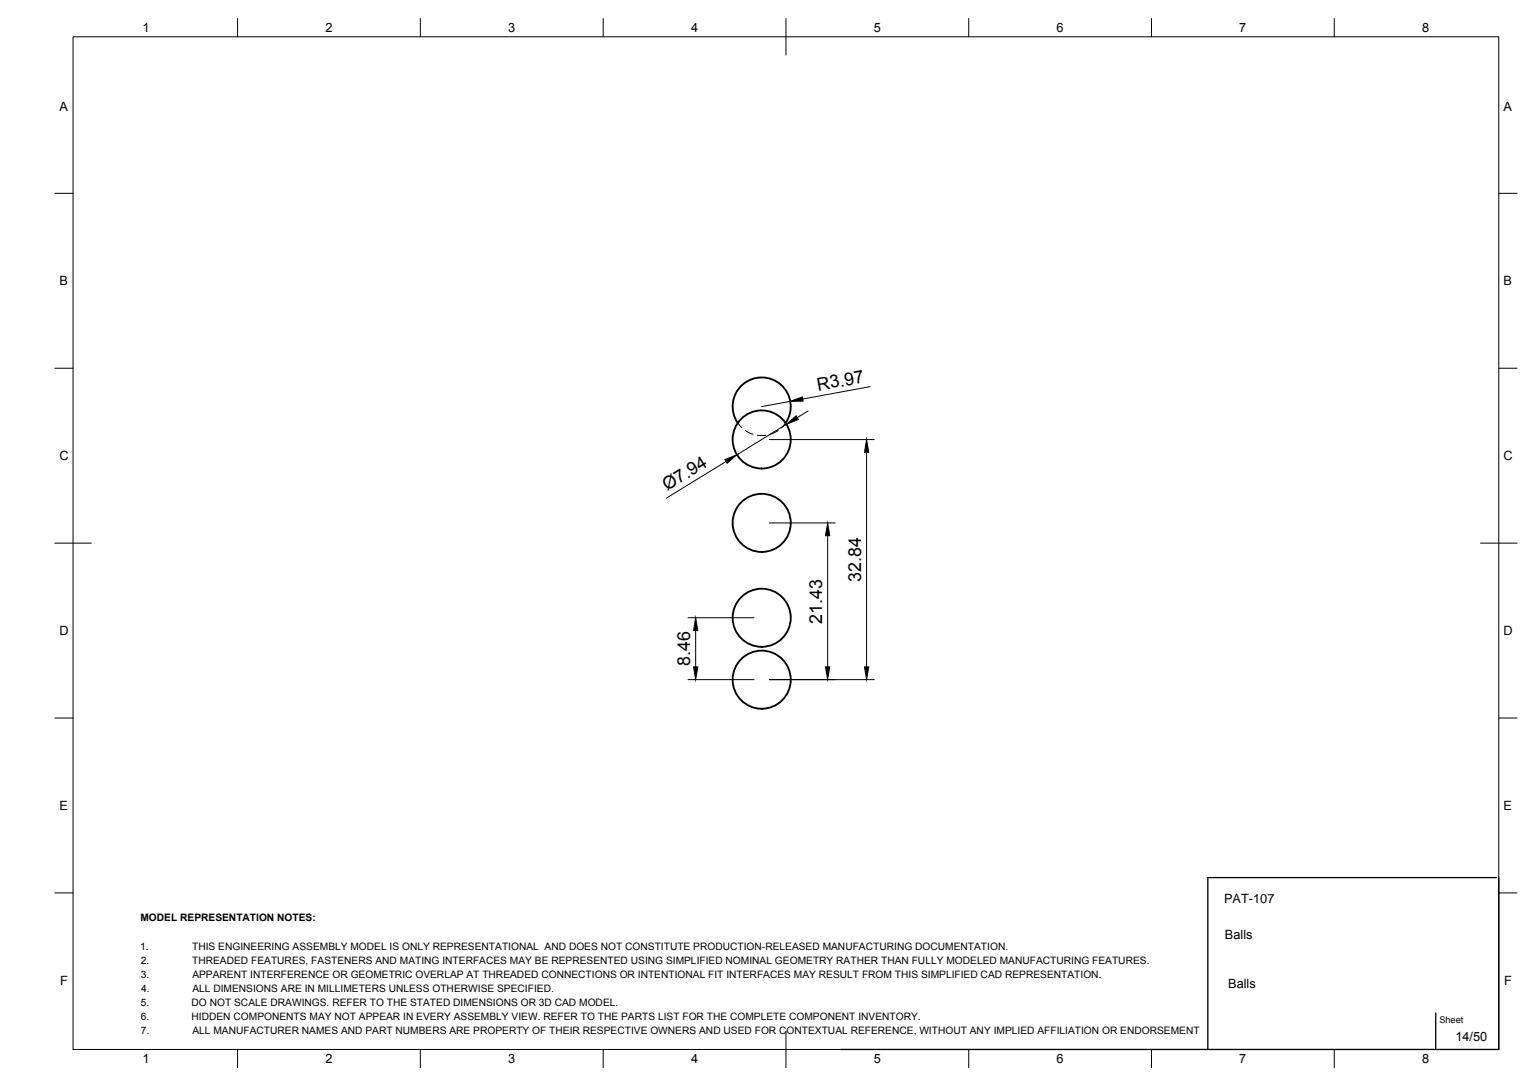
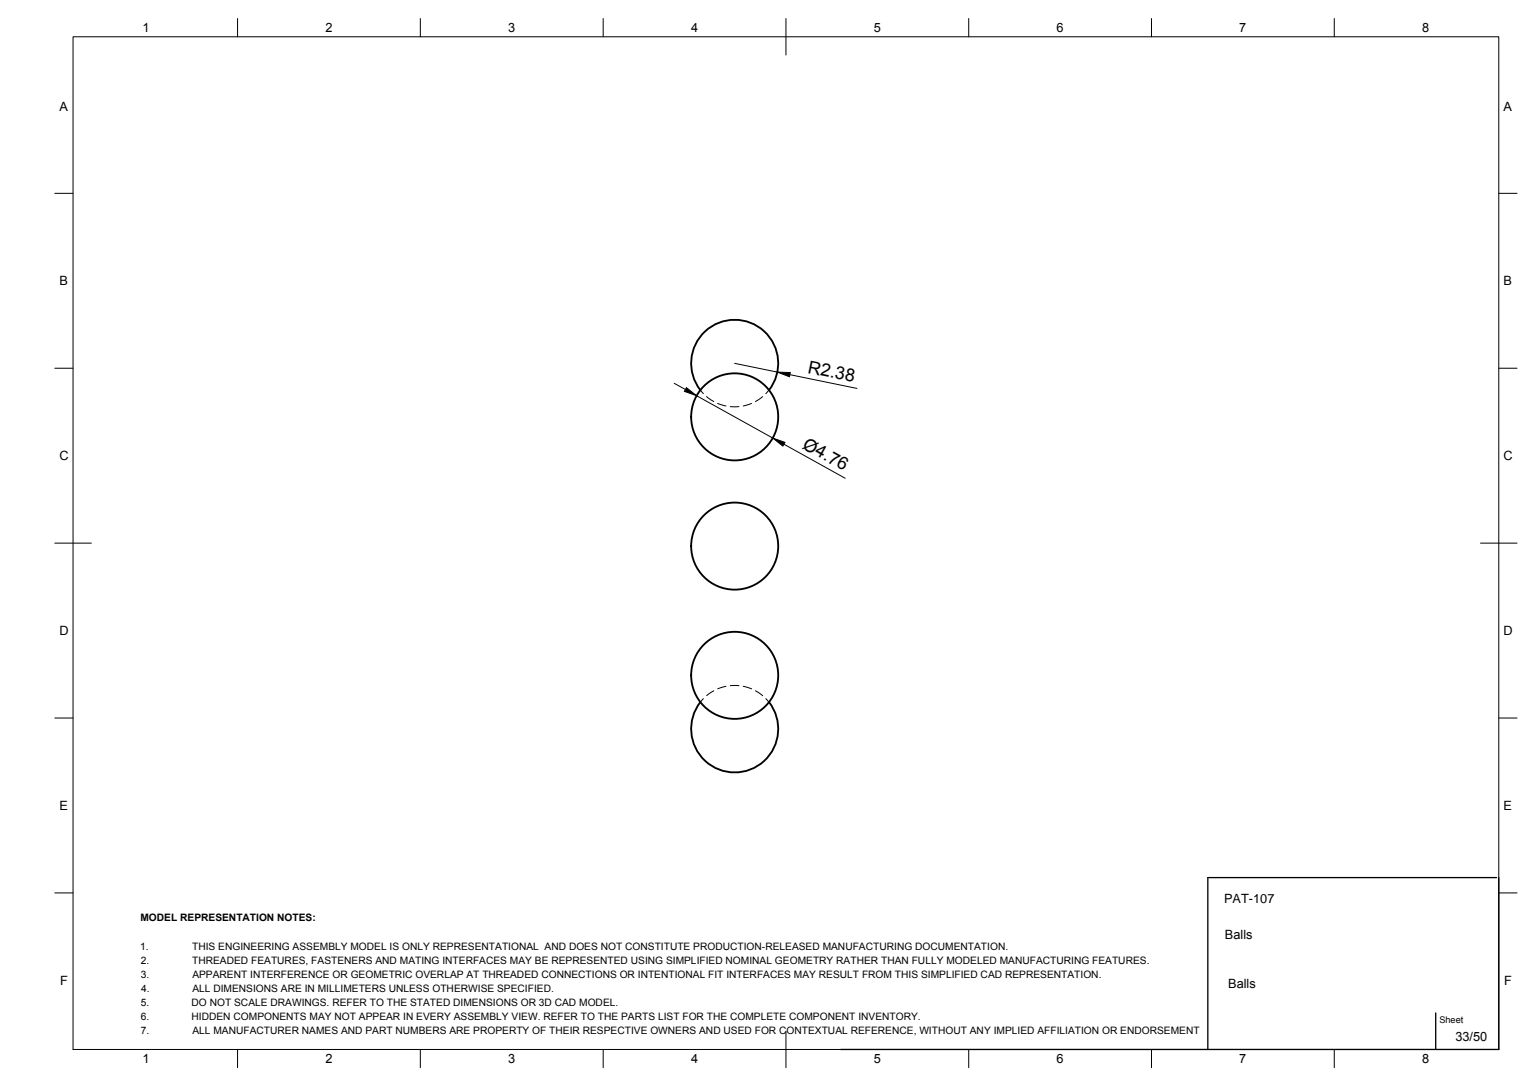
ISO-10303-21;
HEADER;
/* Generated by software containing ST-Developer
 * from STEP Tools, Inc. (www.steptools.com) 
 */

FILE_DESCRIPTION(
/* description */ ('Turntable on roller ring'),
/* implementation_level */ '2;1');

FILE_NAME(
/* name */ 'Balls.step',
/* time_stamp */ '2026-10-28T03:23:59-07:00',
/* author */ (''),
/* organization */ (''),
/* preprocessor_version */ 'ST-DEVELOPER v20.2',
/* originating_system */ 'Autodesk Translation Framework v15.17.0.0',
/* authorisation */ '');

FILE_SCHEMA (('AUTOMOTIVE_DESIGN { 1 0 10303 214 3 1 1 }'));
ENDSEC;

DATA;
#10=MECHANICAL_DESIGN_GEOMETRIC_PRESENTATION_REPRESENTATION('',(#623,#624,#625,#626,#627,#628,#629,#630,#631),#16281);
#438=SPHERICAL_SURFACE('',#9272,0.3969);
#439=SPHERICAL_SURFACE('',#9274,0.3969);
#440=SPHERICAL_SURFACE('',#9276,0.3969);
#441=SPHERICAL_SURFACE('',#9278,0.3969);
#442=SPHERICAL_SURFACE('',#9280,0.3969);
#443=SPHERICAL_SURFACE('',#9282,0.3969);
#444=SPHERICAL_SURFACE('',#9284,0.3969);
#445=SPHERICAL_SURFACE('',#9286,0.3969);
#446=SPHERICAL_SURFACE('',#9288,0.3969);
#513=SHAPE_REPRESENTATION_RELATIONSHIP('SRR','None',#16528,#568);
#568=ADVANCED_BREP_SHAPE_REPRESENTATION('',(#694,#695,#696,#697,#698,#699,
#700,#701,#702),#16222);
#623=STYLED_ITEM('',(#16932),#694);
#624=STYLED_ITEM('',(#16932),#695);
#625=STYLED_ITEM('',(#16932),#696);
#626=STYLED_ITEM('',(#16932),#697);
#627=STYLED_ITEM('',(#16932),#698);
#628=STYLED_ITEM('',(#16932),#699);
#629=STYLED_ITEM('',(#16932),#700);
#630=STYLED_ITEM('',(#16932),#701);
#631=STYLED_ITEM('',(#16932),#702);
#694=MANIFOLD_SOLID_BREP('Body1',#8365);
#695=MANIFOLD_SOLID_BREP('Body2',#8366);
#696=MANIFOLD_SOLID_BREP('Body3',#8367);
#697=MANIFOLD_SOLID_BREP('Body4',#8368);
#698=MANIFOLD_SOLID_BREP('Body5',#8369);
#699=MANIFOLD_SOLID_BREP('Body6',#8370);
#700=MANIFOLD_SOLID_BREP('Body7',#8371);
#701=MANIFOLD_SOLID_BREP('Body8',#8372);
#702=MANIFOLD_SOLID_BREP('Body9',#8373);
#1348=FACE_OUTER_BOUND('',#1924,.T.);
#1349=FACE_OUTER_BOUND('',#1925,.T.);
#1350=FACE_OUTER_BOUND('',#1926,.T.);
#1351=FACE_OUTER_BOUND('',#1927,.T.);
#1352=FACE_OUTER_BOUND('',#1928,.T.);
#1353=FACE_OUTER_BOUND('',#1929,.T.);
#1354=FACE_OUTER_BOUND('',#1930,.T.);
#1355=FACE_OUTER_BOUND('',#1931,.T.);
#1356=FACE_OUTER_BOUND('',#1932,.T.);
#1924=EDGE_LOOP('',(#6083,#6084));
#1925=EDGE_LOOP('',(#6085,#6086));
#1926=EDGE_LOOP('',(#6087,#6088));
#1927=EDGE_LOOP('',(#6089,#6090));
#1928=EDGE_LOOP('',(#6091,#6092));
#1929=EDGE_LOOP('',(#6093,#6094));
#1930=EDGE_LOOP('',(#6095,#6096));
#1931=EDGE_LOOP('',(#6097,#6098));
#1932=EDGE_LOOP('',(#6099,#6100));
#3583=CIRCLE('',#9273,0.3969);
#3584=CIRCLE('',#9275,0.3969);
#3585=CIRCLE('',#9277,0.3969);
#3586=CIRCLE('',#9279,0.3969);
#3587=CIRCLE('',#9281,0.3969);
#3588=CIRCLE('',#9283,0.3969);
#3589=CIRCLE('',#9285,0.3969);
#3590=CIRCLE('',#9287,0.3969);
#3591=CIRCLE('',#9289,0.3969);
#4087=VERTEX_POINT('',#13469);
#4088=VERTEX_POINT('',#13470);
#4089=VERTEX_POINT('',#13473);
#4090=VERTEX_POINT('',#13474);
#4091=VERTEX_POINT('',#13477);
#4092=VERTEX_POINT('',#13478);
#4093=VERTEX_POINT('',#13481);
#4094=VERTEX_POINT('',#13482);
#4095=VERTEX_POINT('',#13485);
#4096=VERTEX_POINT('',#13486);
#4097=VERTEX_POINT('',#13489);
#4098=VERTEX_POINT('',#13490);
#4099=VERTEX_POINT('',#13493);
#4100=VERTEX_POINT('',#13494);
#4101=VERTEX_POINT('',#13497);
#4102=VERTEX_POINT('',#13498);
#4103=VERTEX_POINT('',#13501);
#4104=VERTEX_POINT('',#13502);
#4852=EDGE_CURVE('',#4087,#4088,#3583,.T.);
#4853=EDGE_CURVE('',#4089,#4090,#3584,.T.);
#4854=EDGE_CURVE('',#4091,#4092,#3585,.T.);
#4855=EDGE_CURVE('',#4093,#4094,#3586,.T.);
#4856=EDGE_CURVE('',#4095,#4096,#3587,.T.);
#4857=EDGE_CURVE('',#4097,#4098,#3588,.T.);
#4858=EDGE_CURVE('',#4099,#4100,#3589,.T.);
#4859=EDGE_CURVE('',#4101,#4102,#3590,.T.);
#4860=EDGE_CURVE('',#4103,#4104,#3591,.T.);
#6083=ORIENTED_EDGE('',*,*,#4852,.T.);
#6084=ORIENTED_EDGE('',*,*,#4852,.F.);
#6085=ORIENTED_EDGE('',*,*,#4853,.T.);
#6086=ORIENTED_EDGE('',*,*,#4853,.F.);
#6087=ORIENTED_EDGE('',*,*,#4854,.T.);
#6088=ORIENTED_EDGE('',*,*,#4854,.F.);
#6089=ORIENTED_EDGE('',*,*,#4855,.T.);
#6090=ORIENTED_EDGE('',*,*,#4855,.F.);
#6091=ORIENTED_EDGE('',*,*,#4856,.T.);
#6092=ORIENTED_EDGE('',*,*,#4856,.F.);
#6093=ORIENTED_EDGE('',*,*,#4857,.T.);
#6094=ORIENTED_EDGE('',*,*,#4857,.F.);
#6095=ORIENTED_EDGE('',*,*,#4858,.T.);
#6096=ORIENTED_EDGE('',*,*,#4858,.F.);
#6097=ORIENTED_EDGE('',*,*,#4859,.T.);
#6098=ORIENTED_EDGE('',*,*,#4859,.F.);
#6099=ORIENTED_EDGE('',*,*,#4860,.T.);
#6100=ORIENTED_EDGE('',*,*,#4860,.F.);
#7951=ADVANCED_FACE('',(#1348),#438,.T.);
#7952=ADVANCED_FACE('',(#1349),#439,.T.);
#7953=ADVANCED_FACE('',(#1350),#440,.T.);
#7954=ADVANCED_FACE('',(#1351),#441,.T.);
#7955=ADVANCED_FACE('',(#1352),#442,.T.);
#7956=ADVANCED_FACE('',(#1353),#443,.T.);
#7957=ADVANCED_FACE('',(#1354),#444,.T.);
#7958=ADVANCED_FACE('',(#1355),#445,.T.);
#7959=ADVANCED_FACE('',(#1356),#446,.T.);
#8365=CLOSED_SHELL('',(#7951));
#8366=CLOSED_SHELL('',(#7952));
#8367=CLOSED_SHELL('',(#7953));
#8368=CLOSED_SHELL('',(#7954));
#8369=CLOSED_SHELL('',(#7955));
#8370=CLOSED_SHELL('',(#7956));
#8371=CLOSED_SHELL('',(#7957));
#8372=CLOSED_SHELL('',(#7958));
#8373=CLOSED_SHELL('',(#7959));
#9271=AXIS2_PLACEMENT_3D('',#13467,#10757,#10758);
#9272=AXIS2_PLACEMENT_3D('',#13468,#10759,#10760);
#9273=AXIS2_PLACEMENT_3D('',#13471,#10761,#10762);
#9274=AXIS2_PLACEMENT_3D('',#13472,#10763,#10764);
#9275=AXIS2_PLACEMENT_3D('',#13475,#10765,#10766);
#9276=AXIS2_PLACEMENT_3D('',#13476,#10767,#10768);
#9277=AXIS2_PLACEMENT_3D('',#13479,#10769,#10770);
#9278=AXIS2_PLACEMENT_3D('',#13480,#10771,#10772);
#9279=AXIS2_PLACEMENT_3D('',#13483,#10773,#10774);
#9280=AXIS2_PLACEMENT_3D('',#13484,#10775,#10776);
#9281=AXIS2_PLACEMENT_3D('',#13487,#10777,#10778);
#9282=AXIS2_PLACEMENT_3D('',#13488,#10779,#10780);
#9283=AXIS2_PLACEMENT_3D('',#13491,#10781,#10782);
#9284=AXIS2_PLACEMENT_3D('',#13492,#10783,#10784);
#9285=AXIS2_PLACEMENT_3D('',#13495,#10785,#10786);
#9286=AXIS2_PLACEMENT_3D('',#13496,#10787,#10788);
#9287=AXIS2_PLACEMENT_3D('',#13499,#10789,#10790);
#9288=AXIS2_PLACEMENT_3D('',#13500,#10791,#10792);
#9289=AXIS2_PLACEMENT_3D('',#13503,#10793,#10794);
#10757=DIRECTION('axis',(0.,0.,1.));
#10758=DIRECTION('refdir',(1.,0.,0.));
#10759=DIRECTION('center_axis',(0.,0.,1.));
#10760=DIRECTION('ref_axis',(1.,0.,0.));
#10761=DIRECTION('center_axis',(1.22464679914735E-16,-1.,0.));
#10762=DIRECTION('ref_axis',(-1.,-1.22464679914735E-16,0.));
#10763=DIRECTION('center_axis',(0.642787609686539,0.,0.766044443118978));
#10764=DIRECTION('ref_axis',(0.766044443118978,0.,-0.642787609686539));
#10765=DIRECTION('center_axis',(9.38133875270273E-17,-1.,-7.87187788734199E-17));
#10766=DIRECTION('ref_axis',(-0.766044443118978,-1.22464679914735E-16,0.642787609686539));
#10767=DIRECTION('center_axis',(0.984807753012208,0.,0.173648177666931));
#10768=DIRECTION('ref_axis',(0.17364817766693,0.,-0.984807753012208));
#10769=DIRECTION('center_axis',(2.12657684957577E-17,-1.,-1.2060416625019E-16));
#10770=DIRECTION('ref_axis',(-0.17364817766693,-1.22464679914735E-16,0.984807753012208));
#10771=DIRECTION('center_axis',(0.866025403784439,0.,-0.5));
#10772=DIRECTION('ref_axis',(-0.5,0.,-0.866025403784439));
#10773=DIRECTION('center_axis',(-6.12323399573676E-17,-1.,-1.06057523872491E-16));
#10774=DIRECTION('ref_axis',(0.5,-1.22464679914735E-16,0.866025403784439));
#10775=DIRECTION('center_axis',(0.342020143325669,0.,-0.939692620785908));
#10776=DIRECTION('ref_axis',(-0.939692620785908,0.,-0.342020143325669));
#10777=DIRECTION('center_axis',(-1.15079156022785E-16,-1.,-4.18853873767699E-17));
#10778=DIRECTION('ref_axis',(0.939692620785908,-1.22464679914735E-16,0.342020143325669));
#10779=DIRECTION('center_axis',(-0.342020143325669,0.,-0.939692620785908));
#10780=DIRECTION('ref_axis',(-0.939692620785909,0.,0.342020143325669));
#10781=DIRECTION('center_axis',(-1.15079156022785E-16,-1.,4.18853873767699E-17));
#10782=DIRECTION('ref_axis',(0.939692620785908,-1.22464679914735E-16,-0.342020143325669));
#10783=DIRECTION('center_axis',(-0.866025403784438,0.,-0.5));
#10784=DIRECTION('ref_axis',(-0.5,0.,0.866025403784438));
#10785=DIRECTION('center_axis',(-6.12323399573677E-17,-1.,1.06057523872491E-16));
#10786=DIRECTION('ref_axis',(0.5,-1.22464679914735E-16,-0.866025403784438));
#10787=DIRECTION('center_axis',(-0.984807753012208,0.,0.17364817766693));
#10788=DIRECTION('ref_axis',(0.17364817766693,0.,0.984807753012208));
#10789=DIRECTION('center_axis',(2.12657684957577E-17,-1.,1.2060416625019E-16));
#10790=DIRECTION('ref_axis',(-0.17364817766693,-1.22464679914735E-16,-0.984807753012208));
#10791=DIRECTION('center_axis',(-0.64278760968654,0.,0.766044443118978));
#10792=DIRECTION('ref_axis',(0.766044443118978,0.,0.64278760968654));
#10793=DIRECTION('center_axis',(9.38133875270273E-17,-1.,7.87187788734199E-17));
#10794=DIRECTION('ref_axis',(-0.766044443118978,-1.22464679914735E-16,-0.64278760968654));
#13467=CARTESIAN_POINT('',(0.,0.,0.));
#13468=CARTESIAN_POINT('Origin',(1.925,0.,0.));
#13469=CARTESIAN_POINT('',(1.925,-2.97627328869245E-33,0.3969));
#13470=CARTESIAN_POINT('',(1.925,-2.97627328869245E-33,-0.3969));
#13471=CARTESIAN_POINT('Origin',(1.925,0.,0.));
#13472=CARTESIAN_POINT('Origin',(1.47463555300403,0.,-1.23736614864659));
#13473=CARTESIAN_POINT('',(1.72975795528862,-2.97627328869245E-33,-0.933323109172666));
#13474=CARTESIAN_POINT('',(1.21951315071945,-2.97627328869245E-33,-1.54140918812051));
#13475=CARTESIAN_POINT('Origin',(1.47463555300403,0.,-1.23736614864659));
#13476=CARTESIAN_POINT('Origin',(0.334272742008841,0.,-1.8957549245485));
#13477=CARTESIAN_POINT('',(0.725142939179386,1.05214622327121E-34,-1.8268339628325));
#13478=CARTESIAN_POINT('',(-0.0565974551617042,-6.05776119971203E-33,-1.96467588626451));
#13479=CARTESIAN_POINT('Origin',(0.334272742008841,0.,-1.8957549245485));
#13480=CARTESIAN_POINT('Origin',(-0.9625,0.,-1.66709890228504));
#13481=CARTESIAN_POINT('',(-0.618774517237956,-2.97627328869245E-33,-1.86554890228504));
#13482=CARTESIAN_POINT('',(-1.30622548276204,-2.97627328869245E-33,-1.46864890228504));
#13483=CARTESIAN_POINT('Origin',(-0.9625,0.,-1.66709890228504));
#13484=CARTESIAN_POINT('Origin',(-1.80890829501287,0.,-0.658388775901913));
#13485=CARTESIAN_POINT('',(-1.67316050012692,1.05214622327121E-34,-1.03135277709184));
#13486=CARTESIAN_POINT('',(-1.94465608989883,-6.05776119971203E-33,-0.285424774711986));
#13487=CARTESIAN_POINT('Origin',(-1.80890829501287,0.,-0.658388775901913));
#13488=CARTESIAN_POINT('Origin',(-1.80890829501287,0.,0.658388775901912));
#13489=CARTESIAN_POINT('',(-1.94465608989883,-9.13924911073161E-33,0.285424774711985));
#13490=CARTESIAN_POINT('',(-1.67316050012692,3.1867025333467E-33,1.03135277709184));
#13491=CARTESIAN_POINT('Origin',(-1.80890829501287,0.,0.658388775901912));
#13492=CARTESIAN_POINT('Origin',(-0.962500000000001,0.,1.66709890228504));
#13493=CARTESIAN_POINT('',(-1.30622548276204,-2.97627328869245E-33,1.46864890228504));
#13494=CARTESIAN_POINT('',(-0.618774517237957,-2.97627328869245E-33,1.86554890228504));
#13495=CARTESIAN_POINT('Origin',(-0.962500000000001,0.,1.66709890228504));
#13496=CARTESIAN_POINT('Origin',(0.33427274200884,0.,1.8957549245485));
#13497=CARTESIAN_POINT('',(-0.0565974551617051,-2.97627328869245E-33,1.96467588626451));
#13498=CARTESIAN_POINT('',(0.725142939179386,-2.97627328869245E-33,1.8268339628325));
#13499=CARTESIAN_POINT('Origin',(0.33427274200884,0.,1.8957549245485));
#13500=CARTESIAN_POINT('Origin',(1.47463555300403,0.,1.23736614864659));
#13501=CARTESIAN_POINT('',(1.21951315071944,-6.05776119971203E-33,1.54140918812051));
#13502=CARTESIAN_POINT('',(1.72975795528862,1.05214622327122E-34,0.933323109172667));
#13503=CARTESIAN_POINT('Origin',(1.47463555300403,0.,1.23736614864659));
#16153=UNCERTAINTY_MEASURE_WITH_UNIT(LENGTH_MEASURE(0.001),#16282,
'DISTANCE_ACCURACY_VALUE',
'Maximum model space distance between geometric entities at asserted c
onnectivities');
#16212=UNCERTAINTY_MEASURE_WITH_UNIT(LENGTH_MEASURE(0.001),#16282,
'DISTANCE_ACCURACY_VALUE',
'Maximum model space distance between geometric entities at asserted c
onnectivities');
#16222=(
GEOMETRIC_REPRESENTATION_CONTEXT(3)
GLOBAL_UNCERTAINTY_ASSIGNED_CONTEXT((#16153))
GLOBAL_UNIT_ASSIGNED_CONTEXT((#16282,#16284,#16285))
REPRESENTATION_CONTEXT('','3D')
);
#16281=(
GEOMETRIC_REPRESENTATION_CONTEXT(3)
GLOBAL_UNCERTAINTY_ASSIGNED_CONTEXT((#16212))
GLOBAL_UNIT_ASSIGNED_CONTEXT((#16282,#16284,#16285))
REPRESENTATION_CONTEXT('','3D')
);
#16282=(
LENGTH_UNIT()
NAMED_UNIT(*)
SI_UNIT(.CENTI.,.METRE.)
);
#16284=(
NAMED_UNIT(*)
PLANE_ANGLE_UNIT()
SI_UNIT($,.RADIAN.)
);
#16285=(
NAMED_UNIT(*)
SI_UNIT($,.STERADIAN.)
SOLID_ANGLE_UNIT()
);
#16295=SHAPE_DEFINITION_REPRESENTATION(#16363,#16528);
#16363=PRODUCT_DEFINITION_SHAPE('',$,#16597);
#16528=SHAPE_REPRESENTATION('',(#9271),#16222);
#16587=PRODUCT_DEFINITION_CONTEXT('part definition',#16793,'design');
#16597=PRODUCT_DEFINITION('Balls','Balls',#16665,#16587);
#16665=PRODUCT_DEFINITION_FORMATION('',$,#16804);
#16793=APPLICATION_CONTEXT(
'Core Data for Automotive Mechanical Design Process');
#16794=PRODUCT_CONTEXT('part definition',#16793,'mechanical');
#16804=PRODUCT('Balls','Balls','Balls',(#16794));
#16926=COLOUR_RGB('Grey',0.48,0.52,0.57);
#16927=FILL_AREA_STYLE_COLOUR('',#16926);
#16928=FILL_AREA_STYLE('',(#16927));
#16929=SURFACE_STYLE_FILL_AREA(#16928);
#16930=SURFACE_SIDE_STYLE('',(#16929));
#16931=SURFACE_STYLE_USAGE(.BOTH.,#16930);
#16932=PRESENTATION_STYLE_ASSIGNMENT((#16931));
ENDSEC;
END-ISO-10303-21;
